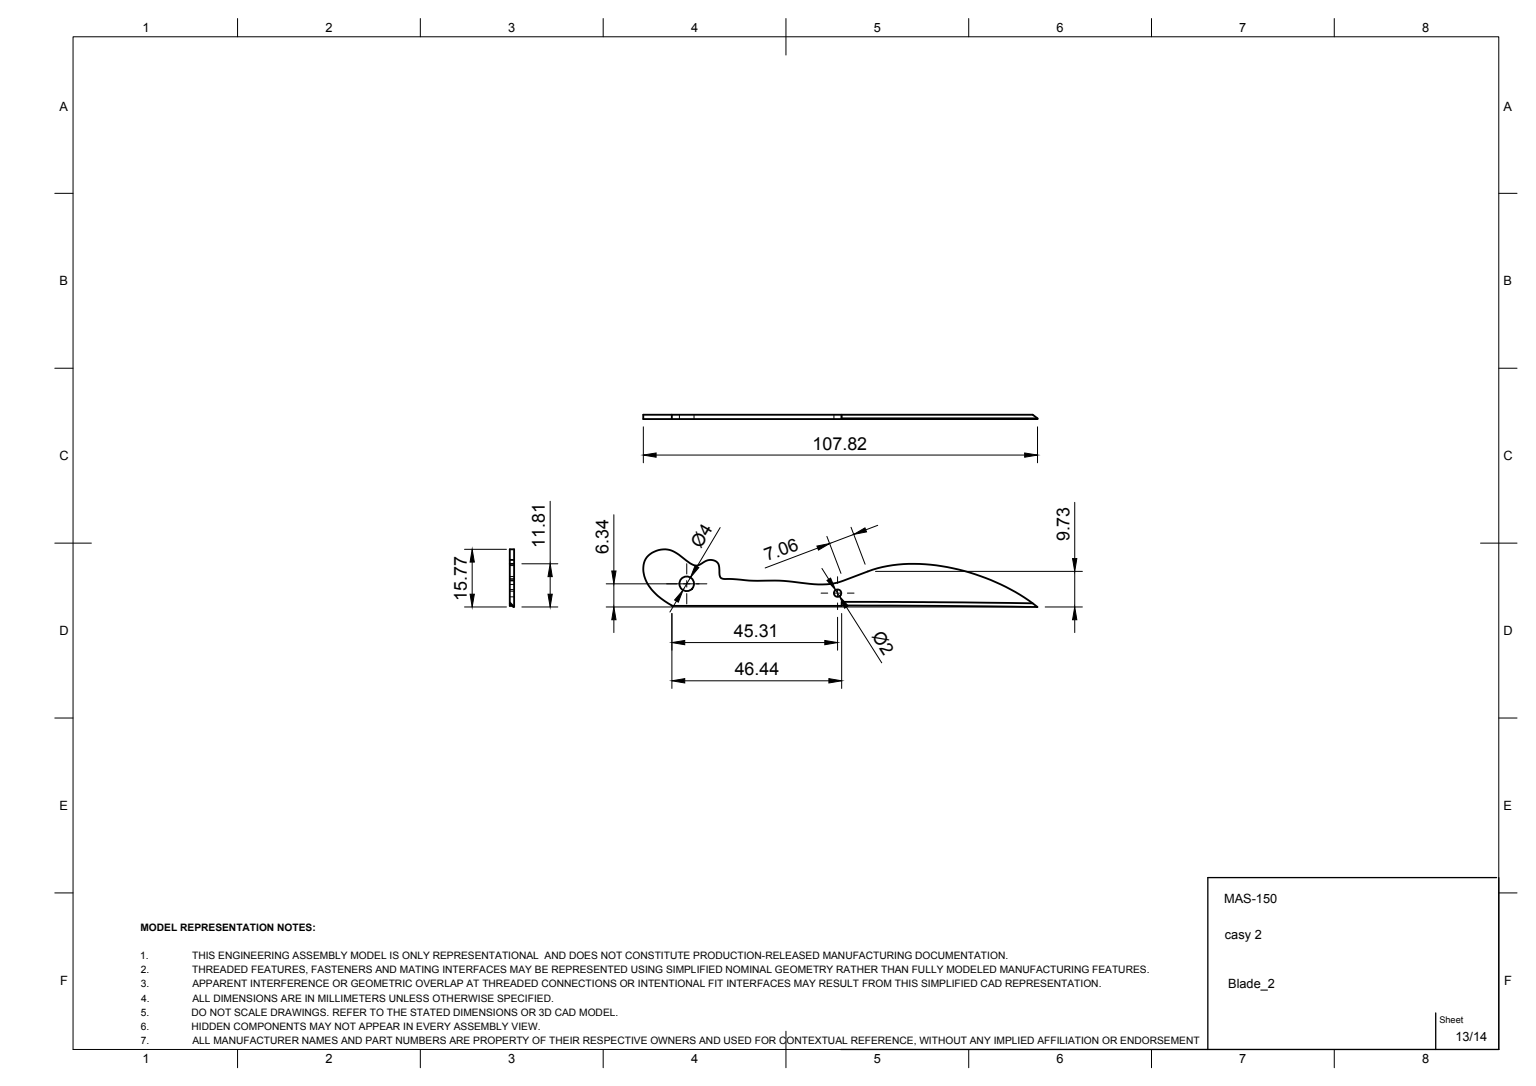
ISO-10303-21;
HEADER;
/* Generated by software containing ST-Developer
 * from STEP Tools, Inc. (www.steptools.com) 
 */

FILE_DESCRIPTION(
/* description */ ('STEP AP203'),
/* implementation_level */ '2;1');

FILE_NAME(
/* name */ 'Blade_2.step',
/* time_stamp */ '2026-11-08T21:40:52-08:00',
/* author */ (''),
/* organization */ (''),
/* preprocessor_version */ 'ST-DEVELOPER v20.2',
/* originating_system */ 'Autodesk Translation Framework v15.17.0.0',
/* authorisation */ '');

FILE_SCHEMA (('AUTOMOTIVE_DESIGN { 1 0 10303 214 3 1 1 }'));
ENDSEC;

DATA;
#10=MECHANICAL_DESIGN_GEOMETRIC_PRESENTATION_REPRESENTATION('',(#187),#12137);
#114=B_SPLINE_CURVE_WITH_KNOTS('',3,(#5044,#5045,#5046,#5047),
 .UNSPECIFIED.,.F.,.F.,(4,4),(0.,0.963009819411559),.UNSPECIFIED.);
#115=B_SPLINE_CURVE_WITH_KNOTS('',3,(#5049,#5050,#5051,#5052,#5053,#5054,
#5055),.UNSPECIFIED.,.F.,.F.,(4,3,4),(-0.194536582159801,-0.0969214136710641,
0.),.UNSPECIFIED.);
#116=B_SPLINE_CURVE_WITH_KNOTS('',3,(#5059,#5060,#5061,#5062),
 .UNSPECIFIED.,.F.,.F.,(4,4),(0.,1.),.UNSPECIFIED.);
#117=B_SPLINE_CURVE_WITH_KNOTS('',3,(#5071,#5072,#5073,#5074,#5075,#5076,
#5077,#5078,#5079,#5080,#5081,#5082,#5083,#5084,#5085,#5086,#5087,#5088,
#5089,#5090,#5091,#5092,#5093,#5094,#5095),.UNSPECIFIED.,.F.,.F.,(4,3,3,
3,3,3,3,3,4),(-4.76083539582986,-4.44733911607309,-4.152057580002,-3.01724680527447,
-2.29831043152851,-1.33769412810892,-0.608765253834458,-0.313488116787147,
0.),.UNSPECIFIED.);
#118=B_SPLINE_CURVE_WITH_KNOTS('',3,(#5131,#5132,#5133,#5134,#5135,#5136,
#5137,#5138,#5139,#5140,#5141,#5142,#5143,#5144,#5145),.UNSPECIFIED.,.F.,
 .F.,(4,1,1,1,1,1,1,1,1,1,1,1,4),(0.,0.157038713621339,0.211241890914945,
0.295200207692272,0.373845032775918,0.419097916699999,0.461946250305228,
0.500883855221145,0.554258304196424,0.580360336370224,0.654376236660092,
0.774520045331176,1.),.UNSPECIFIED.);
#119=B_SPLINE_CURVE_WITH_KNOTS('',3,(#5149,#5150,#5151,#5152,#5153,#5154,
#5155,#5156,#5157,#5158,#5159,#5160,#5161,#5162,#5163),.UNSPECIFIED.,.F.,
 .F.,(4,1,1,1,1,1,1,1,1,1,1,1,4),(0.,0.157038713621339,0.211241890914945,
0.295200207692272,0.373845032775918,0.419097916699999,0.461946250305228,
0.500883855221145,0.554258304196424,0.580360336370224,0.654376236660092,
0.774520045331176,1.),.UNSPECIFIED.);
#120=B_SPLINE_CURVE_WITH_KNOTS('',3,(#5178,#5179,#5180,#5181,#5182,#5183),
 .UNSPECIFIED.,.F.,.F.,(4,2,4),(1.00000017285152E-6,4.02327180930654,8.26259118342642),
 .UNSPECIFIED.);
#152=B_SPLINE_SURFACE_WITH_KNOTS('',3,1,((#5034,#5035),(#5036,#5037),(#5038,
#5039),(#5040,#5041)),.UNSPECIFIED.,.F.,.F.,.F.,(4,4),(2,2),(0.,1.),(0.,
0.1728),.UNSPECIFIED.);
#153=B_SPLINE_SURFACE_WITH_KNOTS('',2,1,((#5064,#5065),(#5066,#5067),(#5068,
#5069)),.UNSPECIFIED.,.F.,.F.,.F.,(3,3),(2,2),(0.,1.),(0.,0.0288000000000019),
 .UNSPECIFIED.);
#154=B_SPLINE_SURFACE_WITH_KNOTS('',3,1,((#5099,#5100),(#5101,#5102),(#5103,
#5104),(#5105,#5106),(#5107,#5108),(#5109,#5110),(#5111,#5112),(#5113,#5114),
(#5115,#5116),(#5117,#5118),(#5119,#5120),(#5121,#5122),(#5123,#5124),(#5125,
#5126),(#5127,#5128)),.UNSPECIFIED.,.F.,.F.,.F.,(4,1,1,1,1,1,1,1,1,1,1,
1,4),(2,2),(0.,0.157038713621339,0.211241890914945,0.295200207692272,0.373845032775918,
0.419097916699999,0.461946250305228,0.500883855221145,0.554258304196424,
0.580360336370224,0.654376236660092,0.774520045331176,1.),(0.,0.1728),
 .UNSPECIFIED.);
#155=B_SPLINE_SURFACE_WITH_KNOTS('',1,3,((#5193,#5194,#5195,#5196,#5197,
#5198,#5199,#5200,#5201,#5202,#5203,#5204,#5205,#5206,#5207,#5208,#5209,
#5210,#5211,#5212,#5213,#5214,#5215,#5216,#5217,#5218,#5219,#5220,#5221,
#5222),(#5223,#5224,#5225,#5226,#5227,#5228,#5229,#5230,#5231,#5232,#5233,
#5234,#5235,#5236,#5237,#5238,#5239,#5240,#5241,#5242,#5243,#5244,#5245,
#5246,#5247,#5248,#5249,#5250,#5251,#5252)),.UNSPECIFIED.,.F.,.F.,.F.,(2,
2),(4,2,2,2,2,2,2,2,2,2,2,2,2,2,4),(-6.70767833503595E-6,1.),(0.0508986734324183,
0.0527402705950223,0.0545818677576262,0.058265062082834,0.0619482564080419,
0.0656314507332498,0.0729978393836655,0.0803642280340812,0.0877306166844969,
0.0950970053349126,0.0987801996601205,0.102463393985328,0.106146588310536,
0.10798818547314,0.109829782635744),.UNSPECIFIED.);
#165=SHAPE_REPRESENTATION_RELATIONSHIP('SRR','None',#12189,#176);
#176=ADVANCED_BREP_SHAPE_REPRESENTATION('',(#198),#12130);
#187=STYLED_ITEM('',(#12253),#198);
#198=MANIFOLD_SOLID_BREP('Body1',#1832);
#215=FACE_BOUND('',#660,.T.);
#216=FACE_BOUND('',#661,.T.);
#217=FACE_BOUND('',#663,.T.);
#218=FACE_BOUND('',#664,.T.);
#248=PLANE('',#2030);
#249=PLANE('',#2031);
#250=PLANE('',#2032);
#251=PLANE('',#2033);
#252=PLANE('',#2034);
#253=PLANE('',#2035);
#318=LINE('',#5026,#412);
#319=LINE('',#5032,#413);
#320=LINE('',#5057,#414);
#321=LINE('',#5063,#415);
#322=LINE('',#5097,#416);
#323=LINE('',#5147,#417);
#324=LINE('',#5164,#418);
#325=LINE('',#5166,#419);
#326=LINE('',#5167,#420);
#327=LINE('',#5170,#421);
#328=LINE('',#5172,#422);
#329=LINE('',#5173,#423);
#330=LINE('',#5177,#424);
#331=LINE('',#5185,#425);
#332=LINE('',#5186,#426);
#333=LINE('',#5188,#427);
#334=LINE('',#5189,#428);
#335=LINE('',#5191,#429);
#412=VECTOR('',#2330,2.00000000000001);
#413=VECTOR('',#2337,1.);
#414=VECTOR('',#2340,1000.);
#415=VECTOR('',#2341,1000.);
#416=VECTOR('',#2342,1000.);
#417=VECTOR('',#2345,1000.);
#418=VECTOR('',#2346,1000.);
#419=VECTOR('',#2349,10.);
#420=VECTOR('',#2350,10.);
#421=VECTOR('',#2353,1000.);
#422=VECTOR('',#2354,1000.);
#423=VECTOR('',#2355,1000.);
#424=VECTOR('',#2358,1000.);
#425=VECTOR('',#2359,1000.);
#426=VECTOR('',#2360,1000.);
#427=VECTOR('',#2363,10.);
#428=VECTOR('',#2364,1000.);
#429=VECTOR('',#2367,1000.);
#473=CYLINDRICAL_SURFACE('',#2023,2.00000000000001);
#474=CYLINDRICAL_SURFACE('',#2026,1.);
#533=FACE_OUTER_BOUND('',#653,.T.);
#534=FACE_OUTER_BOUND('',#654,.T.);
#535=FACE_OUTER_BOUND('',#655,.T.);
#536=FACE_OUTER_BOUND('',#656,.T.);
#537=FACE_OUTER_BOUND('',#657,.T.);
#538=FACE_OUTER_BOUND('',#658,.T.);
#539=FACE_OUTER_BOUND('',#659,.T.);
#540=FACE_OUTER_BOUND('',#662,.T.);
#541=FACE_OUTER_BOUND('',#665,.T.);
#542=FACE_OUTER_BOUND('',#666,.T.);
#543=FACE_OUTER_BOUND('',#667,.T.);
#544=FACE_OUTER_BOUND('',#668,.T.);
#653=EDGE_LOOP('',(#1425,#1426,#1427,#1428));
#654=EDGE_LOOP('',(#1429,#1430,#1431,#1432));
#655=EDGE_LOOP('',(#1433,#1434,#1435,#1436,#1437));
#656=EDGE_LOOP('',(#1438,#1439,#1440,#1441));
#657=EDGE_LOOP('',(#1442,#1443,#1444,#1445));
#658=EDGE_LOOP('',(#1446,#1447,#1448,#1449));
#659=EDGE_LOOP('',(#1450,#1451,#1452,#1453,#1454,#1455,#1456));
#660=EDGE_LOOP('',(#1457));
#661=EDGE_LOOP('',(#1458));
#662=EDGE_LOOP('',(#1459,#1460,#1461,#1462,#1463,#1464,#1465));
#663=EDGE_LOOP('',(#1466));
#664=EDGE_LOOP('',(#1467));
#665=EDGE_LOOP('',(#1468,#1469,#1470,#1471,#1472));
#666=EDGE_LOOP('',(#1473,#1474,#1475,#1476));
#667=EDGE_LOOP('',(#1477,#1478,#1479,#1480));
#668=EDGE_LOOP('',(#1481,#1482,#1483,#1484));
#763=CIRCLE('',#2024,2.00000000000001);
#764=CIRCLE('',#2025,2.00000000000001);
#765=CIRCLE('',#2027,1.);
#766=CIRCLE('',#2028,1.);
#767=CIRCLE('',#2029,3471.58024051075);
#890=VERTEX_POINT('',#5023);
#891=VERTEX_POINT('',#5025);
#892=VERTEX_POINT('',#5029);
#893=VERTEX_POINT('',#5031);
#894=VERTEX_POINT('',#5042);
#895=VERTEX_POINT('',#5043);
#896=VERTEX_POINT('',#5048);
#897=VERTEX_POINT('',#5056);
#898=VERTEX_POINT('',#5058);
#899=VERTEX_POINT('',#5070);
#900=VERTEX_POINT('',#5096);
#901=VERTEX_POINT('',#5129);
#902=VERTEX_POINT('',#5130);
#903=VERTEX_POINT('',#5146);
#904=VERTEX_POINT('',#5148);
#905=VERTEX_POINT('',#5169);
#906=VERTEX_POINT('',#5171);
#907=VERTEX_POINT('',#5175);
#908=VERTEX_POINT('',#5176);
#909=VERTEX_POINT('',#5184);
#1082=EDGE_CURVE('',#890,#890,#763,.T.);
#1083=EDGE_CURVE('',#890,#891,#318,.T.);
#1084=EDGE_CURVE('',#891,#891,#764,.T.);
#1085=EDGE_CURVE('',#892,#892,#765,.T.);
#1086=EDGE_CURVE('',#892,#893,#319,.T.);
#1087=EDGE_CURVE('',#893,#893,#766,.T.);
#1088=EDGE_CURVE('',#894,#895,#114,.T.);
#1089=EDGE_CURVE('',#895,#896,#115,.T.);
#1090=EDGE_CURVE('',#897,#896,#320,.T.);
#1091=EDGE_CURVE('',#898,#897,#116,.T.);
#1092=EDGE_CURVE('',#898,#894,#321,.T.);
#1093=EDGE_CURVE('',#896,#899,#117,.T.);
#1094=EDGE_CURVE('',#900,#899,#322,.T.);
#1095=EDGE_CURVE('',#897,#900,#767,.T.);
#1096=EDGE_CURVE('',#901,#902,#118,.T.);
#1097=EDGE_CURVE('',#903,#902,#323,.T.);
#1098=EDGE_CURVE('',#904,#903,#119,.T.);
#1099=EDGE_CURVE('',#904,#901,#324,.T.);
#1100=EDGE_CURVE('',#902,#894,#325,.T.);
#1101=EDGE_CURVE('',#903,#898,#326,.T.);
#1102=EDGE_CURVE('',#905,#900,#327,.T.);
#1103=EDGE_CURVE('',#906,#905,#328,.T.);
#1104=EDGE_CURVE('',#906,#904,#329,.T.);
#1105=EDGE_CURVE('',#907,#908,#330,.T.);
#1106=EDGE_CURVE('',#908,#895,#120,.T.);
#1107=EDGE_CURVE('',#909,#901,#331,.T.);
#1108=EDGE_CURVE('',#907,#909,#332,.T.);
#1109=EDGE_CURVE('',#899,#908,#333,.T.);
#1110=EDGE_CURVE('',#905,#907,#334,.T.);
#1111=EDGE_CURVE('',#909,#906,#335,.T.);
#1425=ORIENTED_EDGE('',*,*,#1082,.F.);
#1426=ORIENTED_EDGE('',*,*,#1083,.T.);
#1427=ORIENTED_EDGE('',*,*,#1084,.T.);
#1428=ORIENTED_EDGE('',*,*,#1083,.F.);
#1429=ORIENTED_EDGE('',*,*,#1085,.F.);
#1430=ORIENTED_EDGE('',*,*,#1086,.T.);
#1431=ORIENTED_EDGE('',*,*,#1087,.T.);
#1432=ORIENTED_EDGE('',*,*,#1086,.F.);
#1433=ORIENTED_EDGE('',*,*,#1088,.T.);
#1434=ORIENTED_EDGE('',*,*,#1089,.T.);
#1435=ORIENTED_EDGE('',*,*,#1090,.F.);
#1436=ORIENTED_EDGE('',*,*,#1091,.F.);
#1437=ORIENTED_EDGE('',*,*,#1092,.T.);
#1438=ORIENTED_EDGE('',*,*,#1090,.T.);
#1439=ORIENTED_EDGE('',*,*,#1093,.T.);
#1440=ORIENTED_EDGE('',*,*,#1094,.F.);
#1441=ORIENTED_EDGE('',*,*,#1095,.F.);
#1442=ORIENTED_EDGE('',*,*,#1096,.T.);
#1443=ORIENTED_EDGE('',*,*,#1097,.F.);
#1444=ORIENTED_EDGE('',*,*,#1098,.F.);
#1445=ORIENTED_EDGE('',*,*,#1099,.T.);
#1446=ORIENTED_EDGE('',*,*,#1100,.T.);
#1447=ORIENTED_EDGE('',*,*,#1092,.F.);
#1448=ORIENTED_EDGE('',*,*,#1101,.F.);
#1449=ORIENTED_EDGE('',*,*,#1097,.T.);
#1450=ORIENTED_EDGE('',*,*,#1091,.T.);
#1451=ORIENTED_EDGE('',*,*,#1095,.T.);
#1452=ORIENTED_EDGE('',*,*,#1102,.F.);
#1453=ORIENTED_EDGE('',*,*,#1103,.F.);
#1454=ORIENTED_EDGE('',*,*,#1104,.T.);
#1455=ORIENTED_EDGE('',*,*,#1098,.T.);
#1456=ORIENTED_EDGE('',*,*,#1101,.T.);
#1457=ORIENTED_EDGE('',*,*,#1084,.F.);
#1458=ORIENTED_EDGE('',*,*,#1087,.F.);
#1459=ORIENTED_EDGE('',*,*,#1105,.T.);
#1460=ORIENTED_EDGE('',*,*,#1106,.T.);
#1461=ORIENTED_EDGE('',*,*,#1088,.F.);
#1462=ORIENTED_EDGE('',*,*,#1100,.F.);
#1463=ORIENTED_EDGE('',*,*,#1096,.F.);
#1464=ORIENTED_EDGE('',*,*,#1107,.F.);
#1465=ORIENTED_EDGE('',*,*,#1108,.F.);
#1466=ORIENTED_EDGE('',*,*,#1082,.T.);
#1467=ORIENTED_EDGE('',*,*,#1085,.T.);
#1468=ORIENTED_EDGE('',*,*,#1094,.T.);
#1469=ORIENTED_EDGE('',*,*,#1109,.T.);
#1470=ORIENTED_EDGE('',*,*,#1105,.F.);
#1471=ORIENTED_EDGE('',*,*,#1110,.F.);
#1472=ORIENTED_EDGE('',*,*,#1102,.T.);
#1473=ORIENTED_EDGE('',*,*,#1099,.F.);
#1474=ORIENTED_EDGE('',*,*,#1104,.F.);
#1475=ORIENTED_EDGE('',*,*,#1111,.F.);
#1476=ORIENTED_EDGE('',*,*,#1107,.T.);
#1477=ORIENTED_EDGE('',*,*,#1103,.T.);
#1478=ORIENTED_EDGE('',*,*,#1110,.T.);
#1479=ORIENTED_EDGE('',*,*,#1108,.T.);
#1480=ORIENTED_EDGE('',*,*,#1111,.T.);
#1481=ORIENTED_EDGE('',*,*,#1089,.F.);
#1482=ORIENTED_EDGE('',*,*,#1106,.F.);
#1483=ORIENTED_EDGE('',*,*,#1109,.F.);
#1484=ORIENTED_EDGE('',*,*,#1093,.F.);
#1761=ADVANCED_FACE('',(#533),#473,.F.);
#1762=ADVANCED_FACE('',(#534),#474,.F.);
#1763=ADVANCED_FACE('',(#535),#152,.F.);
#1764=ADVANCED_FACE('',(#536),#153,.F.);
#1765=ADVANCED_FACE('',(#537),#154,.F.);
#1766=ADVANCED_FACE('',(#538),#248,.F.);
#1767=ADVANCED_FACE('',(#539,#215,#216),#249,.T.);
#1768=ADVANCED_FACE('',(#540,#217,#218),#250,.F.);
#1769=ADVANCED_FACE('',(#541),#251,.F.);
#1770=ADVANCED_FACE('',(#542),#252,.F.);
#1771=ADVANCED_FACE('',(#543),#253,.T.);
#1772=ADVANCED_FACE('',(#544),#155,.T.);
#1832=CLOSED_SHELL('',(#1761,#1762,#1763,#1764,#1765,#1766,#1767,#1768,
#1769,#1770,#1771,#1772));
#2022=AXIS2_PLACEMENT_3D('',#5021,#2324,#2325);
#2023=AXIS2_PLACEMENT_3D('',#5022,#2326,#2327);
#2024=AXIS2_PLACEMENT_3D('',#5024,#2328,#2329);
#2025=AXIS2_PLACEMENT_3D('',#5027,#2331,#2332);
#2026=AXIS2_PLACEMENT_3D('',#5028,#2333,#2334);
#2027=AXIS2_PLACEMENT_3D('',#5030,#2335,#2336);
#2028=AXIS2_PLACEMENT_3D('',#5033,#2338,#2339);
#2029=AXIS2_PLACEMENT_3D('',#5098,#2343,#2344);
#2030=AXIS2_PLACEMENT_3D('',#5165,#2347,#2348);
#2031=AXIS2_PLACEMENT_3D('',#5168,#2351,#2352);
#2032=AXIS2_PLACEMENT_3D('',#5174,#2356,#2357);
#2033=AXIS2_PLACEMENT_3D('',#5187,#2361,#2362);
#2034=AXIS2_PLACEMENT_3D('',#5190,#2365,#2366);
#2035=AXIS2_PLACEMENT_3D('',#5192,#2368,#2369);
#2324=DIRECTION('axis',(0.,0.,1.));
#2325=DIRECTION('refdir',(1.,0.,0.));
#2326=DIRECTION('center_axis',(0.,1.,0.));
#2327=DIRECTION('ref_axis',(0.,0.,1.));
#2328=DIRECTION('center_axis',(0.,1.,0.));
#2329=DIRECTION('ref_axis',(0.,0.,1.));
#2330=DIRECTION('',(0.,1.,0.));
#2331=DIRECTION('center_axis',(0.,1.,0.));
#2332=DIRECTION('ref_axis',(0.,0.,1.));
#2333=DIRECTION('center_axis',(0.,1.,0.));
#2334=DIRECTION('ref_axis',(2.168404344971E-16,0.,1.));
#2335=DIRECTION('center_axis',(0.,1.,0.));
#2336=DIRECTION('ref_axis',(2.168404344971E-16,0.,1.));
#2337=DIRECTION('',(0.,1.,0.));
#2338=DIRECTION('center_axis',(0.,1.,0.));
#2339=DIRECTION('ref_axis',(2.168404344971E-16,0.,1.));
#2340=DIRECTION('',(0.,-1.,0.));
#2341=DIRECTION('',(0.,-1.,0.));
#2342=DIRECTION('',(0.,-1.,0.));
#2343=DIRECTION('center_axis',(0.,-1.,0.));
#2344=DIRECTION('ref_axis',(0.873216452631512,0.,-0.487332562890721));
#2345=DIRECTION('',(0.,-1.,0.));
#2346=DIRECTION('',(0.,-1.,0.));
#2347=DIRECTION('center_axis',(-0.989219464793322,0.,0.146440603911665));
#2348=DIRECTION('ref_axis',(0.146440603911665,0.,0.989219464793322));
#2349=DIRECTION('',(-0.146440603911672,0.,-0.989219464793321));
#2350=DIRECTION('',(-0.146440603911672,0.,-0.989219464793321));
#2351=DIRECTION('center_axis',(0.,1.,0.));
#2352=DIRECTION('ref_axis',(1.11022302462515E-16,0.,1.));
#2353=DIRECTION('',(0.873216508553205,0.,-0.487332462688615));
#2354=DIRECTION('',(-0.487332462688615,0.,-0.873216508553205));
#2355=DIRECTION('',(0.873216508553205,0.,-0.487332462688615));
#2356=DIRECTION('center_axis',(0.,1.,0.));
#2357=DIRECTION('ref_axis',(1.11022302462515E-16,0.,1.));
#2358=DIRECTION('',(0.873216508553205,0.,-0.487332462688615));
#2359=DIRECTION('',(0.873216508553205,0.,-0.487332462688615));
#2360=DIRECTION('',(0.487332462688615,0.,0.873216508553205));
#2361=DIRECTION('center_axis',(0.487332462688615,0.,0.873216508553205));
#2362=DIRECTION('ref_axis',(0.873216508553205,0.,-0.487332462688615));
#2363=DIRECTION('',(0.6174573145645,-0.707106781319327,-0.344596088925887));
#2364=DIRECTION('',(0.,-1.,0.));
#2365=DIRECTION('center_axis',(-0.487332462688615,0.,-0.873216508553205));
#2366=DIRECTION('ref_axis',(-0.873216508553205,0.,0.487332462688615));
#2367=DIRECTION('',(0.,1.,0.));
#2368=DIRECTION('center_axis',(-0.873216508553205,0.,0.487332462688615));
#2369=DIRECTION('ref_axis',(0.487332462688615,0.,0.873216508553205));
#5021=CARTESIAN_POINT('',(0.,0.,0.));
#5022=CARTESIAN_POINT('Origin',(21.1914505799844,-0.000524999999999484,
34.7829861880462));
#5023=CARTESIAN_POINT('',(21.1914505799844,0.,32.7829861880461));
#5024=CARTESIAN_POINT('Origin',(21.1914505799844,0.,34.7829861880462));
#5025=CARTESIAN_POINT('',(21.1914505799844,1.2,32.7829861880461));
#5026=CARTESIAN_POINT('',(21.1914505799844,-0.000524999999999484,32.7829861880462));
#5027=CARTESIAN_POINT('Origin',(21.1914505799844,1.2,34.7829861880462));
#5028=CARTESIAN_POINT('Origin',(-1.14649136662881,0.,0.));
#5029=CARTESIAN_POINT('',(-1.14649136662881,0.,-1.));
#5030=CARTESIAN_POINT('Origin',(-1.14649136662881,0.,0.));
#5031=CARTESIAN_POINT('',(-1.14649136662881,1.2,-1.));
#5032=CARTESIAN_POINT('',(-1.14649136662881,0.,-1.));
#5033=CARTESIAN_POINT('Origin',(-1.14649136662881,1.2,0.));
#5034=CARTESIAN_POINT('Ctrl Pts',(0.0163039410302629,1.2,-10.1188450599643));
#5035=CARTESIAN_POINT('Ctrl Pts',(0.0163039410302629,-0.528,-10.1188450599643));
#5036=CARTESIAN_POINT('Ctrl Pts',(-2.21904904761523,1.2,-25.218855767281));
#5037=CARTESIAN_POINT('Ctrl Pts',(-2.21904904761523,-0.528,-25.218855767281));
#5038=CARTESIAN_POINT('Ctrl Pts',(-17.3117222200821,1.2,-40.3484435255013));
#5039=CARTESIAN_POINT('Ctrl Pts',(-17.3117222200821,-0.528,-40.3484435255013));
#5040=CARTESIAN_POINT('Ctrl Pts',(-31.0970400923937,1.2,-45.9093754426411));
#5041=CARTESIAN_POINT('Ctrl Pts',(-31.0970400923937,-0.528,-45.9093754426411));
#5042=CARTESIAN_POINT('',(0.0163039410302629,0.,-10.1188450599643));
#5043=CARTESIAN_POINT('',(-29.5626263532375,-7.98607492925424E-16,-45.2534839938841));
#5044=CARTESIAN_POINT('Ctrl Pts',(0.0163039410302629,0.,-10.1188450599643));
#5045=CARTESIAN_POINT('Ctrl Pts',(-2.13636293688632,0.,-24.66030364433));
#5046=CARTESIAN_POINT('Ctrl Pts',(-16.2127531376322,0.,-39.2291916281846));
#5047=CARTESIAN_POINT('Ctrl Pts',(-29.5626263532375,0.,-45.253483993884));
#5048=CARTESIAN_POINT('',(-31.0970400928039,0.999993661824606,-45.9093754428066));
#5049=CARTESIAN_POINT('Ctrl Pts',(-29.5626263532375,-1.80411241501588E-15,
-45.2534839938841));
#5050=CARTESIAN_POINT('Ctrl Pts',(-29.8188688224744,0.163986041940123,-45.3691165190969));
#5051=CARTESIAN_POINT('Ctrl Pts',(-30.075375785987,0.329632644340004,-45.4818409421178));
#5052=CARTESIAN_POINT('Ctrl Pts',(-30.3320199519673,0.496887461248793,-45.5915431280263));
#5053=CARTESIAN_POINT('Ctrl Pts',(-30.5868401378292,0.66295359163677,-45.7004656562119));
#5054=CARTESIAN_POINT('Ctrl Pts',(-30.8418789960871,0.830662075864011,-45.806444665302));
#5055=CARTESIAN_POINT('Ctrl Pts',(-31.0970400923937,0.999993661442804,-45.9093754426411));
#5056=CARTESIAN_POINT('',(-31.0970400923937,1.2,-45.9093754426411));
#5057=CARTESIAN_POINT('',(-31.0970400923937,1.2,-45.9093754426411));
#5058=CARTESIAN_POINT('',(0.0163039410302629,1.2,-10.1188450599643));
#5059=CARTESIAN_POINT('Ctrl Pts',(0.0163039410302629,1.2,-10.1188450599643));
#5060=CARTESIAN_POINT('Ctrl Pts',(-2.21904904761523,1.2,-25.218855767281));
#5061=CARTESIAN_POINT('Ctrl Pts',(-17.3117222200821,1.2,-40.3484435255013));
#5062=CARTESIAN_POINT('Ctrl Pts',(-31.0970400923937,1.2,-45.9093754426411));
#5063=CARTESIAN_POINT('',(0.0163039410302629,1.2,-10.1188450599643));
#5064=CARTESIAN_POINT('Ctrl Pts',(-31.0970400923937,1.2,-45.9093754426411));
#5065=CARTESIAN_POINT('Ctrl Pts',(-31.0970400923937,0.911999999999981,-45.9093754426411));
#5066=CARTESIAN_POINT('Ctrl Pts',(-17.686844155281,1.2,-22.7283469888476));
#5067=CARTESIAN_POINT('Ctrl Pts',(-17.686844155281,0.911999999999981,-22.7283469888476));
#5068=CARTESIAN_POINT('Ctrl Pts',(-4.63662953841448,1.2,0.655407872751923));
#5069=CARTESIAN_POINT('Ctrl Pts',(-4.63662953841448,0.911999999999981,0.655407872751923));
#5070=CARTESIAN_POINT('',(-4.63662953868546,0.999993660672008,0.655407872945712));
#5071=CARTESIAN_POINT('Ctrl Pts',(-31.0970400923936,0.99999366103201,-45.909375442641));
#5072=CARTESIAN_POINT('Ctrl Pts',(-30.573767819807,0.999956907587257,-45.004840602375));
#5073=CARTESIAN_POINT('Ctrl Pts',(-30.0144098007429,1.00000670634066,-44.0369858115081));
#5074=CARTESIAN_POINT('Ctrl Pts',(-29.4221965441832,1.00000295949628,-43.0109978936339));
#5075=CARTESIAN_POINT('Ctrl Pts',(-28.8643920298385,0.999999430350852,-42.0446218696016));
#5076=CARTESIAN_POINT('Ctrl Pts',(-28.307044239795,0.999999999781451,-41.0779611336147));
#5077=CARTESIAN_POINT('Ctrl Pts',(-27.7501655379961,0.999999999832482,-40.1110370623424));
#5078=CARTESIAN_POINT('Ctrl Pts',(-25.6099980238801,1.0000000000286,-36.3950043261841));
#5079=CARTESIAN_POINT('Ctrl Pts',(-23.476715914865,0.999999999148073,-32.6750077927901));
#5080=CARTESIAN_POINT('Ctrl Pts',(-21.35033689032,0.999999999476567,-28.951076996802));
#5081=CARTESIAN_POINT('Ctrl Pts',(-20.0032125422252,0.999999999684679,-26.5918560921613));
#5082=CARTESIAN_POINT('Ctrl Pts',(-18.6588566071828,1.00000000011496,-24.231052287125));
#5083=CARTESIAN_POINT('Ctrl Pts',(-17.3172728840955,0.999999999975142,-21.8686720102845));
#5084=CARTESIAN_POINT('Ctrl Pts',(-15.5246981252401,0.999999999788324,-18.7121464933104));
#5085=CARTESIAN_POINT('Ctrl Pts',(-13.7370789901641,0.999999998628723,-15.5528175743293));
#5086=CARTESIAN_POINT('Ctrl Pts',(-11.9544155689351,0.999999999319974,-12.390685202677));
#5087=CARTESIAN_POINT('Ctrl Pts',(-10.6017060258834,0.999999999844504,-9.99121563114253));
#5088=CARTESIAN_POINT('Ctrl Pts',(-9.25185160494225,1.00000000000002,-7.5901347140568));
#5089=CARTESIAN_POINT('Ctrl Pts',(-7.90485658637567,1.00000000000003,-5.18745008485492));
#5090=CARTESIAN_POINT('Ctrl Pts',(-7.35921098673439,1.00000000000004,-4.21416193071989));
#5091=CARTESIAN_POINT('Ctrl Pts',(-6.814037789644,0.999999430754603,-3.24061632119799));
#5092=CARTESIAN_POINT('Ctrl Pts',(-6.26933697629459,1.00000296037334,-2.26681326697206));
#5093=CARTESIAN_POINT('Ctrl Pts',(-5.69104217874656,1.00000670767848,-1.23295169325346));
#5094=CARTESIAN_POINT('Ctrl Pts',(-5.14587265802439,0.99995690076854,-0.257068789396161));
#5095=CARTESIAN_POINT('Ctrl Pts',(-4.63662953841449,0.999993659872726,0.655407872751901));
#5096=CARTESIAN_POINT('',(-4.63662953841448,1.2,0.655407872751923));
#5097=CARTESIAN_POINT('',(-4.63662953841448,1.2,0.655407872751923));
#5098=CARTESIAN_POINT('Origin',(-3036.07761218286,1.2,1692.46950376164));
#5099=CARTESIAN_POINT('Ctrl Pts',(17.9965481466234,1.2,41.2101952278912));
#5100=CARTESIAN_POINT('Ctrl Pts',(17.9965481466234,-0.528,41.2101952278912));
#5101=CARTESIAN_POINT('Ctrl Pts',(21.1524317437801,1.2,43.1694484023668));
#5102=CARTESIAN_POINT('Ctrl Pts',(21.1524317437801,-0.528,43.1694484023668));
#5103=CARTESIAN_POINT('Ctrl Pts',(26.9936524453639,1.2,45.5981161424412));
#5104=CARTESIAN_POINT('Ctrl Pts',(26.9936524453639,-0.528,45.5981161424412));
#5105=CARTESIAN_POINT('Ctrl Pts',(33.9307266408316,1.2,41.1415677861088));
#5106=CARTESIAN_POINT('Ctrl Pts',(33.9307266408316,-0.528,41.1415677861088));
#5107=CARTESIAN_POINT('Ctrl Pts',(32.8535862824509,1.2,33.9883280103707));
#5108=CARTESIAN_POINT('Ctrl Pts',(32.8535862824509,-0.528,33.9883280103707));
#5109=CARTESIAN_POINT('Ctrl Pts',(27.9014606940056,1.2,32.3046097776791));
#5110=CARTESIAN_POINT('Ctrl Pts',(27.9014606940056,-0.528,32.3046097776791));
#5111=CARTESIAN_POINT('Ctrl Pts',(23.322809839386,1.2,30.2059351076599));
#5112=CARTESIAN_POINT('Ctrl Pts',(23.322809839386,-0.528,30.2059351076599));
#5113=CARTESIAN_POINT('Ctrl Pts',(24.7202491484524,1.2,26.5916170055359));
#5114=CARTESIAN_POINT('Ctrl Pts',(24.7202491484524,-0.528,26.5916170055359));
#5115=CARTESIAN_POINT('Ctrl Pts',(21.5911557932172,1.2,23.2911168236856));
#5116=CARTESIAN_POINT('Ctrl Pts',(21.5911557932172,-0.528,23.2911168236856));
#5117=CARTESIAN_POINT('Ctrl Pts',(18.2287371224104,1.2,27.0608466969321));
#5118=CARTESIAN_POINT('Ctrl Pts',(18.2287371224104,-0.528,27.0608466969321));
#5119=CARTESIAN_POINT('Ctrl Pts',(16.1921180788491,1.2,22.8319263998159));
#5120=CARTESIAN_POINT('Ctrl Pts',(16.1921180788491,-0.528,22.8319263998159));
#5121=CARTESIAN_POINT('Ctrl Pts',(12.9326029577631,1.2,18.8909674054421));
#5122=CARTESIAN_POINT('Ctrl Pts',(12.9326029577631,-0.528,18.8909674054421));
#5123=CARTESIAN_POINT('Ctrl Pts',(8.48253901799792,1.2,8.87740159675101));
#5124=CARTESIAN_POINT('Ctrl Pts',(8.48253901799792,-0.528,8.87740159675101));
#5125=CARTESIAN_POINT('Ctrl Pts',(1.84058088196348,1.2,2.8000810225724));
#5126=CARTESIAN_POINT('Ctrl Pts',(1.84058088196348,-0.528,2.8000810225724));
#5127=CARTESIAN_POINT('Ctrl Pts',(1.05043439536577,1.2,-3.13320072882459));
#5128=CARTESIAN_POINT('Ctrl Pts',(1.05043439536577,-0.528,-3.13320072882459));
#5129=CARTESIAN_POINT('',(17.9965481466234,0.,41.2101952278912));
#5130=CARTESIAN_POINT('',(1.05043439536577,0.,-3.13320072882459));
#5131=CARTESIAN_POINT('Ctrl Pts',(17.9965481466234,0.,41.2101952278912));
#5132=CARTESIAN_POINT('Ctrl Pts',(21.1524317437801,0.,43.1694484023668));
#5133=CARTESIAN_POINT('Ctrl Pts',(26.9936524453639,0.,45.5981161424412));
#5134=CARTESIAN_POINT('Ctrl Pts',(33.9307266408316,0.,41.1415677861088));
#5135=CARTESIAN_POINT('Ctrl Pts',(32.8535862824509,0.,33.9883280103707));
#5136=CARTESIAN_POINT('Ctrl Pts',(27.9014606940056,0.,32.3046097776791));
#5137=CARTESIAN_POINT('Ctrl Pts',(23.322809839386,0.,30.2059351076599));
#5138=CARTESIAN_POINT('Ctrl Pts',(24.7202491484524,0.,26.5916170055359));
#5139=CARTESIAN_POINT('Ctrl Pts',(21.5911557932172,0.,23.2911168236856));
#5140=CARTESIAN_POINT('Ctrl Pts',(18.2287371224104,0.,27.0608466969321));
#5141=CARTESIAN_POINT('Ctrl Pts',(16.1921180788491,0.,22.8319263998159));
#5142=CARTESIAN_POINT('Ctrl Pts',(12.9326029577631,0.,18.8909674054421));
#5143=CARTESIAN_POINT('Ctrl Pts',(8.48253901799792,0.,8.87740159675101));
#5144=CARTESIAN_POINT('Ctrl Pts',(1.84058088196348,0.,2.8000810225724));
#5145=CARTESIAN_POINT('Ctrl Pts',(1.05043439536577,0.,-3.13320072882459));
#5146=CARTESIAN_POINT('',(1.05043439536577,1.2,-3.13320072882459));
#5147=CARTESIAN_POINT('',(1.05043439536577,1.2,-3.13320072882459));
#5148=CARTESIAN_POINT('',(17.9965481466234,1.2,41.2101952278912));
#5149=CARTESIAN_POINT('Ctrl Pts',(17.9965481466234,1.2,41.2101952278912));
#5150=CARTESIAN_POINT('Ctrl Pts',(21.1524317437801,1.2,43.1694484023668));
#5151=CARTESIAN_POINT('Ctrl Pts',(26.9936524453639,1.2,45.5981161424412));
#5152=CARTESIAN_POINT('Ctrl Pts',(33.9307266408316,1.2,41.1415677861088));
#5153=CARTESIAN_POINT('Ctrl Pts',(32.8535862824509,1.2,33.9883280103707));
#5154=CARTESIAN_POINT('Ctrl Pts',(27.9014606940056,1.2,32.3046097776791));
#5155=CARTESIAN_POINT('Ctrl Pts',(23.322809839386,1.2,30.2059351076599));
#5156=CARTESIAN_POINT('Ctrl Pts',(24.7202491484524,1.2,26.5916170055359));
#5157=CARTESIAN_POINT('Ctrl Pts',(21.5911557932172,1.2,23.2911168236856));
#5158=CARTESIAN_POINT('Ctrl Pts',(18.2287371224104,1.2,27.0608466969321));
#5159=CARTESIAN_POINT('Ctrl Pts',(16.1921180788491,1.2,22.8319263998159));
#5160=CARTESIAN_POINT('Ctrl Pts',(12.9326029577631,1.2,18.8909674054421));
#5161=CARTESIAN_POINT('Ctrl Pts',(8.48253901799792,1.2,8.87740159675101));
#5162=CARTESIAN_POINT('Ctrl Pts',(1.84058088196348,1.2,2.8000810225724));
#5163=CARTESIAN_POINT('Ctrl Pts',(1.05043439536577,1.2,-3.13320072882459));
#5164=CARTESIAN_POINT('',(17.9965481466234,1.2,41.2101952278912));
#5165=CARTESIAN_POINT('Origin',(1.05043439536577,1.2,-3.13320072882459));
#5166=CARTESIAN_POINT('',(1.05043439536577,0.,-3.13320072882459));
#5167=CARTESIAN_POINT('',(1.05043439536577,1.2,-3.13320072882459));
#5168=CARTESIAN_POINT('Origin',(-11.2091312443069,1.2,-31.591264797619));
#5169=CARTESIAN_POINT('',(-4.7239511892698,1.2,0.704141119020785));
#5170=CARTESIAN_POINT('',(-4.7239511892698,1.2,0.704141119020785));
#5171=CARTESIAN_POINT('',(17.9092264957681,1.2,41.2589284741601));
#5172=CARTESIAN_POINT('',(17.9092264957681,1.2,41.2589284741601));
#5173=CARTESIAN_POINT('',(17.9092264957681,1.2,41.2589284741601));
#5174=CARTESIAN_POINT('Origin',(-11.2091312443069,0.,-31.591264797619));
#5175=CARTESIAN_POINT('',(-4.7239511892698,0.,0.704141119020785));
#5176=CARTESIAN_POINT('',(-3.7634185663843,0.,0.168078500190919));
#5177=CARTESIAN_POINT('',(-4.7239511892698,0.,0.704141119020785));
#5178=CARTESIAN_POINT('Ctrl Pts',(-3.7634185663843,0.,0.168078500190915));
#5179=CARTESIAN_POINT('Ctrl Pts',(-10.2994008356464,0.,-11.5423169605017));
#5180=CARTESIAN_POINT('Ctrl Pts',(-12.4600130210599,1.38777878078145E-15,
-15.3418604059716));
#5181=CARTESIAN_POINT('Ctrl Pts',(-20.9163234840607,1.38777878078145E-15,
-30.2298597196315));
#5182=CARTESIAN_POINT('Ctrl Pts',(-25.2491386822615,0.,-37.790624293729));
#5183=CARTESIAN_POINT('Ctrl Pts',(-29.5626263532375,0.,-45.2534839938841));
#5184=CARTESIAN_POINT('',(17.9092264957681,0.,41.2589284741601));
#5185=CARTESIAN_POINT('',(17.9092264957681,0.,41.2589284741601));
#5186=CARTESIAN_POINT('',(-4.7239511892698,0.,0.704141119020785));
#5187=CARTESIAN_POINT('Origin',(-4.7239511892698,1.2,0.704141119020785));
#5188=CARTESIAN_POINT('',(-4.6366323065132,0.99999682993773,0.655409417724869));
#5189=CARTESIAN_POINT('',(-4.7239511892698,1.2,0.704141119020785));
#5190=CARTESIAN_POINT('Origin',(17.9092264957681,0.,41.2589284741601));
#5191=CARTESIAN_POINT('',(17.9092264957681,0.,41.2589284741601));
#5192=CARTESIAN_POINT('Origin',(-3.90169114982751,0.,2.17749062010543));
#5193=CARTESIAN_POINT('Ctrl Pts',(-32.4383859892945,1.00000670767832,-48.2280289443117));
#5194=CARTESIAN_POINT('Ctrl Pts',(-32.1309955518262,1.00000670767832,-47.6966700804449));
#5195=CARTESIAN_POINT('Ctrl Pts',(-31.8236175039076,1.00000670767832,-47.1653405930931));
#5196=CARTESIAN_POINT('Ctrl Pts',(-31.2088118498719,1.00000670767832,-46.1025641123295));
#5197=CARTESIAN_POINT('Ctrl Pts',(-30.9014508032936,1.00000670767832,-45.5713166895576));
#5198=CARTESIAN_POINT('Ctrl Pts',(-29.9800401478882,1.00000670767832,-43.9775269224044));
#5199=CARTESIAN_POINT('Ctrl Pts',(-29.366284226523,1.00000670767832,-42.9145488034795));
#5200=CARTESIAN_POINT('Ctrl Pts',(-28.1399451284085,1.00000670767832,-40.7880674192455));
#5201=CARTESIAN_POINT('Ctrl Pts',(-27.5273384407701,1.00000670767832,-39.7244999614497));
#5202=CARTESIAN_POINT('Ctrl Pts',(-26.3032558235069,1.00000670767832,-37.5967201796819));
#5203=CARTESIAN_POINT('Ctrl Pts',(-25.6917792941021,1.00000670767832,-36.5325068181677));
#5204=CARTESIAN_POINT('Ctrl Pts',(-23.8590452247175,1.00000670767832,-33.3388982832929));
#5205=CARTESIAN_POINT('Ctrl Pts',(-22.6394819645239,1.00000670767832,-31.2085325126316));
#5206=CARTESIAN_POINT('Ctrl Pts',(-20.2048756335948,1.00000670767832,-26.9452159217588));
#5207=CARTESIAN_POINT('Ctrl Pts',(-18.9898323807444,1.00000670767832,-24.8122647858504));
#5208=CARTESIAN_POINT('Ctrl Pts',(-16.5642658874957,1.00000670767832,-20.5437767101294));
#5209=CARTESIAN_POINT('Ctrl Pts',(-15.3537487180158,1.00000670767832,-18.408250451539));
#5210=CARTESIAN_POINT('Ctrl Pts',(-12.9372473733207,1.00000670767832,-14.1346348557454));
#5211=CARTESIAN_POINT('Ctrl Pts',(-11.7312616183177,1.00000670767832,-11.9965427097547));
#5212=CARTESIAN_POINT('Ctrl Pts',(-9.92568646806448,1.00000670767832,-8.78748872799292));
#5213=CARTESIAN_POINT('Ctrl Pts',(-9.32439612554591,1.00000670767832,-7.71748618845371));
#5214=CARTESIAN_POINT('Ctrl Pts',(-8.12295077554065,1.00000670767832,-5.57684403913935));
#5215=CARTESIAN_POINT('Ctrl Pts',(-7.52279589125647,1.00000670767832,-4.50620464856389));
#5216=CARTESIAN_POINT('Ctrl Pts',(-6.32362169657787,1.00000670767832,-2.36428923843985));
#5217=CARTESIAN_POINT('Ctrl Pts',(-5.72456001077879,1.00000670767832,-1.29296148385365));
#5218=CARTESIAN_POINT('Ctrl Pts',(-4.82694628305467,1.00000670767832,0.314352412496741));
#5219=CARTESIAN_POINT('Ctrl Pts',(-4.52786990488178,1.00000670767832,0.850308497929449));
#5220=CARTESIAN_POINT('Ctrl Pts',(-3.92951798462665,1.00000670767832,1.92243654538334));
#5221=CARTESIAN_POINT('Ctrl Pts',(-3.63037981674452,1.00000670767832,2.45844921237444));
#5222=CARTESIAN_POINT('Ctrl Pts',(-3.33122275273957,1.00000670767832,2.99448755773365));
#5223=CARTESIAN_POINT('Ctrl Pts',(-31.5727855656386,0.,-48.7287777056367));
#5224=CARTESIAN_POINT('Ctrl Pts',(-31.2653951281703,0.,-48.1974188417698));
#5225=CARTESIAN_POINT('Ctrl Pts',(-30.9580012389628,0.,-47.666061973265));
#5226=CARTESIAN_POINT('Ctrl Pts',(-30.3432272675049,0.,-46.6033402548073));
#5227=CARTESIAN_POINT('Ctrl Pts',(-30.0358105356997,0.,-46.071996591336));
#5228=CARTESIAN_POINT('Ctrl Pts',(-29.1140850373573,0.,-44.477662286746));
#5229=CARTESIAN_POINT('Ctrl Pts',(-28.5001853221512,0.,-43.4144350187497));
#5230=CARTESIAN_POINT('Ctrl Pts',(-27.2734930129072,0.,-41.2873411637132));
#5231=CARTESIAN_POINT('Ctrl Pts',(-26.6607098789485,0.,-40.2234673714217));
#5232=CARTESIAN_POINT('Ctrl Pts',(-25.4362746895989,0.,-38.0950747259902));
#5233=CARTESIAN_POINT('Ctrl Pts',(-24.8246220342551,0.,-37.0305548350095));
#5234=CARTESIAN_POINT('Ctrl Pts',(-22.9913600686247,0.,-33.8360264209311));
#5235=CARTESIAN_POINT('Ctrl Pts',(-21.7714455193403,1.73472347597681E-15,
-31.7050470091101));
#5236=CARTESIAN_POINT('Ctrl Pts',(-19.336137898936,0.,-27.4405023679293));
#5237=CARTESIAN_POINT('Ctrl Pts',(-18.1207446456488,0.,-25.3069368227818));
#5238=CARTESIAN_POINT('Ctrl Pts',(-15.6944794449877,0.,-21.0372191686235));
#5239=CARTESIAN_POINT('Ctrl Pts',(-14.4836135702811,0.,-18.9010777439119));
#5240=CARTESIAN_POINT('Ctrl Pts',(-12.0664161170873,0.,-14.6262310707415));
#5241=CARTESIAN_POINT('Ctrl Pts',(-10.8600829583573,0.,-12.4875230126863));
#5242=CARTESIAN_POINT('Ctrl Pts',(-9.05398768358211,0.,-9.2775446120943));
#5243=CARTESIAN_POINT('Ctrl Pts',(-8.4525241299626,0.,-8.20723384156397));
#5244=CARTESIAN_POINT('Ctrl Pts',(-7.2507326856024,0.,-6.06597504816851));
#5245=CARTESIAN_POINT('Ctrl Pts',(-6.65040491809978,0.,-4.99502724456632));
#5246=CARTESIAN_POINT('Ctrl Pts',(-5.45088528547934,0.,-2.85249482746024));
#5247=CARTESIAN_POINT('Ctrl Pts',(-4.85168313295727,0.,-1.78091598210246));
#5248=CARTESIAN_POINT('Ctrl Pts',(-3.95376268794949,0.,-0.173052805131788));
#5249=CARTESIAN_POINT('Ctrl Pts',(-3.6546321212938,0.,0.363000394754204));
#5250=CARTESIAN_POINT('Ctrl Pts',(-3.05631103659737,0.,1.43507318544256));
#5251=CARTESIAN_POINT('Ctrl Pts',(-2.75715745093588,0.,1.97111348081644));
#5252=CARTESIAN_POINT('Ctrl Pts',(-2.45800038693092,0.,2.50715182617563));
#12116=UNCERTAINTY_MEASURE_WITH_UNIT(LENGTH_MEASURE(0.01),#12138,
'DISTANCE_ACCURACY_VALUE',
'Maximum model space distance between geometric entities at asserted c
onnectivities');
#12123=UNCERTAINTY_MEASURE_WITH_UNIT(LENGTH_MEASURE(0.01),#12138,
'DISTANCE_ACCURACY_VALUE',
'Maximum model space distance between geometric entities at asserted c
onnectivities');
#12130=(
GEOMETRIC_REPRESENTATION_CONTEXT(3)
GLOBAL_UNCERTAINTY_ASSIGNED_CONTEXT((#12116))
GLOBAL_UNIT_ASSIGNED_CONTEXT((#12138,#12140,#12141))
REPRESENTATION_CONTEXT('','3D')
);
#12137=(
GEOMETRIC_REPRESENTATION_CONTEXT(3)
GLOBAL_UNCERTAINTY_ASSIGNED_CONTEXT((#12123))
GLOBAL_UNIT_ASSIGNED_CONTEXT((#12138,#12140,#12141))
REPRESENTATION_CONTEXT('','3D')
);
#12138=(
LENGTH_UNIT()
NAMED_UNIT(*)
SI_UNIT(.MILLI.,.METRE.)
);
#12140=(
NAMED_UNIT(*)
PLANE_ANGLE_UNIT()
SI_UNIT($,.RADIAN.)
);
#12141=(
NAMED_UNIT(*)
SI_UNIT($,.STERADIAN.)
SOLID_ANGLE_UNIT()
);
#12148=SHAPE_DEFINITION_REPRESENTATION(#12161,#12189);
#12161=PRODUCT_DEFINITION_SHAPE('',$,#12203);
#12189=SHAPE_REPRESENTATION('',(#2022),#12130);
#12196=PRODUCT_DEFINITION_CONTEXT('part definition',#12237,'design');
#12203=PRODUCT_DEFINITION('casy 2','Blade_2',#12216,#12196);
#12216=PRODUCT_DEFINITION_FORMATION('',$,#12245);
#12237=APPLICATION_CONTEXT(
'Core Data for Automotive Mechanical Design Process');
#12238=PRODUCT_CONTEXT('part definition',#12237,'mechanical');
#12245=PRODUCT('casy 2','Blade_2',$,(#12238));
#12253=PRESENTATION_STYLE_ASSIGNMENT((#12255));
#12255=SURFACE_STYLE_USAGE(.BOTH.,#12257);
#12257=SURFACE_SIDE_STYLE('',(#12259));
#12259=SURFACE_STYLE_FILL_AREA(#12261);
#12261=FILL_AREA_STYLE('Opaque(23,69,131)',(#12263));
#12263=FILL_AREA_STYLE_COLOUR('Opaque(23,69,131)',#12265);
#12265=COLOUR_RGB('Opaque(23,69,131)',0.0901960784313725,0.270588235294118,
0.513725490196078);
ENDSEC;
END-ISO-10303-21;
